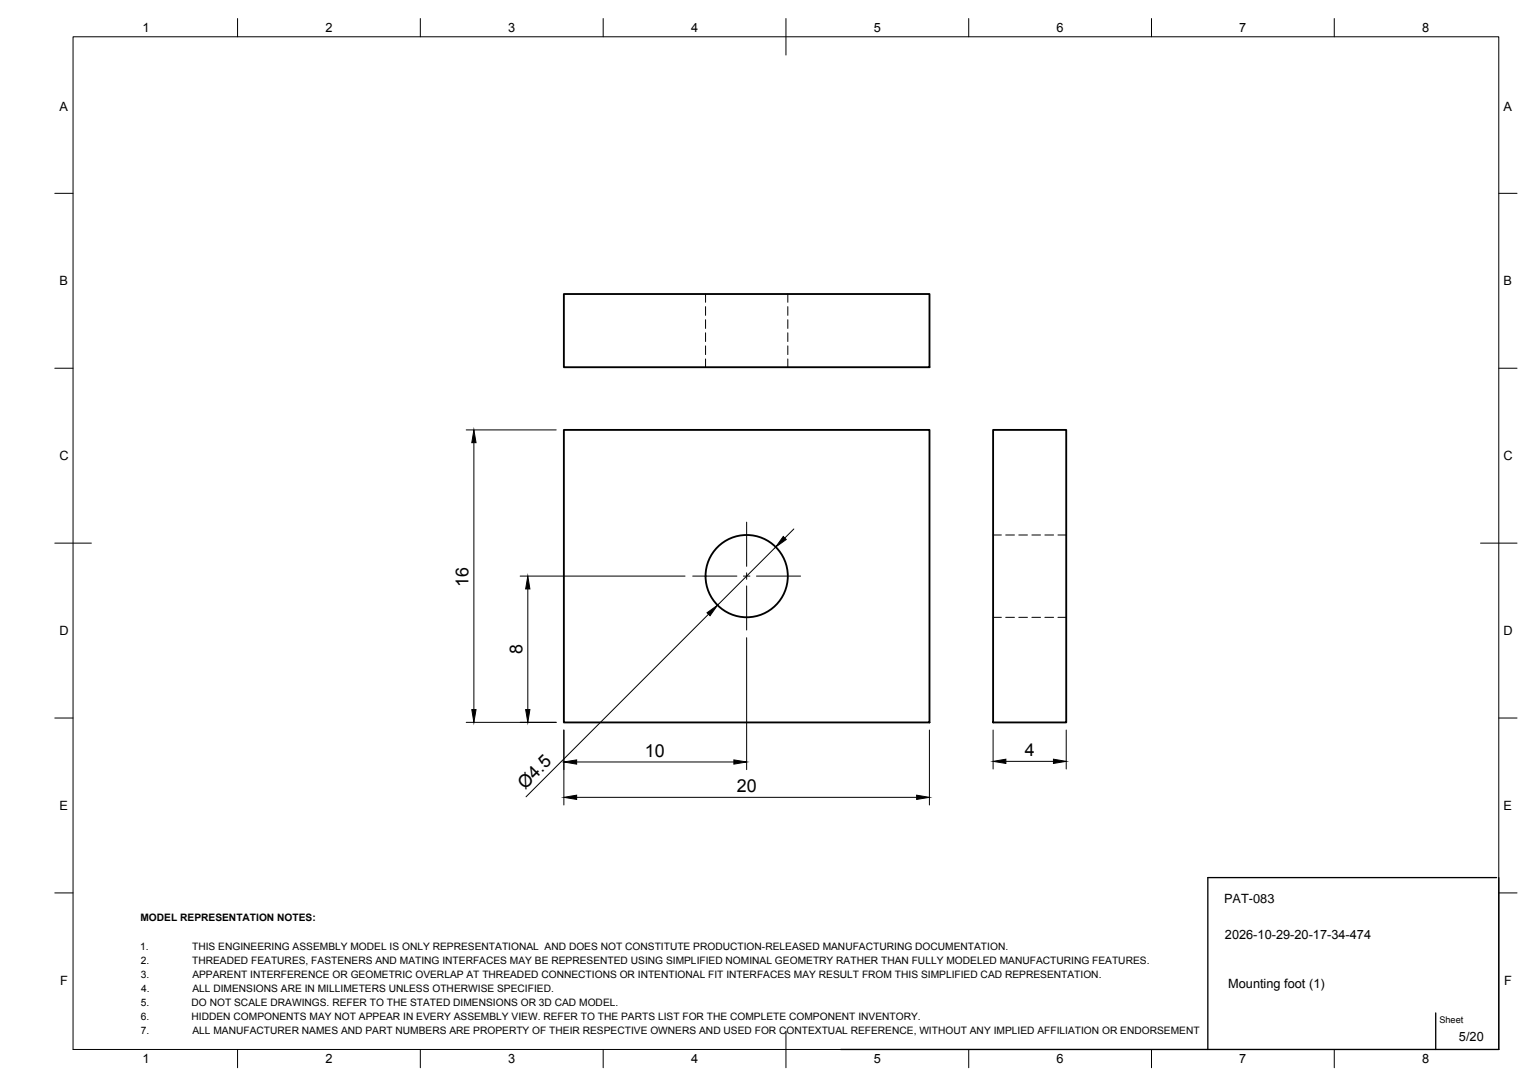
ISO-10303-21;
HEADER;
/* Generated by software containing ST-Developer
 * from STEP Tools, Inc. (www.steptools.com) 
 */

FILE_DESCRIPTION(
/* description */ ('PAT-083'),
/* implementation_level */ '2;1');

FILE_NAME(
/* name */ 'Mounting foot (1).step',
/* time_stamp */ '2026-10-29T20:18:00-07:00',
/* author */ (''),
/* organization */ (''),
/* preprocessor_version */ 'ST-DEVELOPER v20.2',
/* originating_system */ 'Autodesk Translation Framework v15.17.0.0',
/* authorisation */ '');

FILE_SCHEMA (('AUTOMOTIVE_DESIGN { 1 0 10303 214 3 1 1 }'));
ENDSEC;

DATA;
#10=MECHANICAL_DESIGN_GEOMETRIC_PRESENTATION_REPRESENTATION('',(#231),#8428);
#183=SHAPE_REPRESENTATION_RELATIONSHIP('SRR','None',#8517,#207);
#207=ADVANCED_BREP_SHAPE_REPRESENTATION('',(#255),#8406);
#231=STYLED_ITEM('',(#8698),#255);
#255=MANIFOLD_SOLID_BREP('Body1',#3677);
#281=FACE_BOUND('',#755,.T.);
#282=FACE_BOUND('',#757,.T.);
#368=PLANE('',#3994);
#369=PLANE('',#3995);
#370=PLANE('',#3996);
#371=PLANE('',#3997);
#372=PLANE('',#3998);
#373=PLANE('',#3999);
#510=FACE_OUTER_BOUND('',#749,.T.);
#511=FACE_OUTER_BOUND('',#750,.T.);
#512=FACE_OUTER_BOUND('',#751,.T.);
#513=FACE_OUTER_BOUND('',#752,.T.);
#514=FACE_OUTER_BOUND('',#753,.T.);
#515=FACE_OUTER_BOUND('',#754,.T.);
#516=FACE_OUTER_BOUND('',#756,.T.);
#749=EDGE_LOOP('',(#2524,#2525,#2526,#2527));
#750=EDGE_LOOP('',(#2528,#2529,#2530,#2531));
#751=EDGE_LOOP('',(#2532,#2533,#2534,#2535));
#752=EDGE_LOOP('',(#2536,#2537,#2538,#2539));
#753=EDGE_LOOP('',(#2540,#2541,#2542,#2543));
#754=EDGE_LOOP('',(#2544,#2545,#2546,#2547));
#755=EDGE_LOOP('',(#2548));
#756=EDGE_LOOP('',(#2549,#2550,#2551,#2552));
#757=EDGE_LOOP('',(#2553));
#1069=LINE('',#5698,#1313);
#1070=LINE('',#5703,#1314);
#1071=LINE('',#5705,#1315);
#1072=LINE('',#5707,#1316);
#1073=LINE('',#5708,#1317);
#1074=LINE('',#5711,#1318);
#1075=LINE('',#5713,#1319);
#1076=LINE('',#5714,#1320);
#1077=LINE('',#5717,#1321);
#1078=LINE('',#5719,#1322);
#1079=LINE('',#5720,#1323);
#1080=LINE('',#5722,#1324);
#1081=LINE('',#5723,#1325);
#1313=VECTOR('',#4517,0.225);
#1314=VECTOR('',#4522,1.);
#1315=VECTOR('',#4523,1.);
#1316=VECTOR('',#4524,1.);
#1317=VECTOR('',#4525,1.);
#1318=VECTOR('',#4528,1.);
#1319=VECTOR('',#4529,1.);
#1320=VECTOR('',#4530,1.);
#1321=VECTOR('',#4533,1.);
#1322=VECTOR('',#4534,1.);
#1323=VECTOR('',#4535,1.);
#1324=VECTOR('',#4538,1.);
#1325=VECTOR('',#4539,1.);
#1536=CIRCLE('',#3992,0.225);
#1537=CIRCLE('',#3993,0.225);
#1735=VERTEX_POINT('',#5695);
#1736=VERTEX_POINT('',#5697);
#1737=VERTEX_POINT('',#5701);
#1738=VERTEX_POINT('',#5702);
#1739=VERTEX_POINT('',#5704);
#1740=VERTEX_POINT('',#5706);
#1741=VERTEX_POINT('',#5710);
#1742=VERTEX_POINT('',#5712);
#1743=VERTEX_POINT('',#5716);
#1744=VERTEX_POINT('',#5718);
#2038=EDGE_CURVE('',#1735,#1735,#1536,.T.);
#2039=EDGE_CURVE('',#1735,#1736,#1069,.T.);
#2040=EDGE_CURVE('',#1736,#1736,#1537,.T.);
#2041=EDGE_CURVE('',#1737,#1738,#1070,.T.);
#2042=EDGE_CURVE('',#1738,#1739,#1071,.T.);
#2043=EDGE_CURVE('',#1740,#1739,#1072,.T.);
#2044=EDGE_CURVE('',#1737,#1740,#1073,.T.);
#2045=EDGE_CURVE('',#1741,#1737,#1074,.T.);
#2046=EDGE_CURVE('',#1742,#1740,#1075,.T.);
#2047=EDGE_CURVE('',#1741,#1742,#1076,.T.);
#2048=EDGE_CURVE('',#1743,#1741,#1077,.T.);
#2049=EDGE_CURVE('',#1744,#1742,#1078,.T.);
#2050=EDGE_CURVE('',#1743,#1744,#1079,.T.);
#2051=EDGE_CURVE('',#1738,#1743,#1080,.T.);
#2052=EDGE_CURVE('',#1739,#1744,#1081,.T.);
#2524=ORIENTED_EDGE('',*,*,#2038,.F.);
#2525=ORIENTED_EDGE('',*,*,#2039,.T.);
#2526=ORIENTED_EDGE('',*,*,#2040,.F.);
#2527=ORIENTED_EDGE('',*,*,#2039,.F.);
#2528=ORIENTED_EDGE('',*,*,#2041,.T.);
#2529=ORIENTED_EDGE('',*,*,#2042,.T.);
#2530=ORIENTED_EDGE('',*,*,#2043,.F.);
#2531=ORIENTED_EDGE('',*,*,#2044,.F.);
#2532=ORIENTED_EDGE('',*,*,#2045,.T.);
#2533=ORIENTED_EDGE('',*,*,#2044,.T.);
#2534=ORIENTED_EDGE('',*,*,#2046,.F.);
#2535=ORIENTED_EDGE('',*,*,#2047,.F.);
#2536=ORIENTED_EDGE('',*,*,#2048,.T.);
#2537=ORIENTED_EDGE('',*,*,#2047,.T.);
#2538=ORIENTED_EDGE('',*,*,#2049,.F.);
#2539=ORIENTED_EDGE('',*,*,#2050,.F.);
#2540=ORIENTED_EDGE('',*,*,#2051,.T.);
#2541=ORIENTED_EDGE('',*,*,#2050,.T.);
#2542=ORIENTED_EDGE('',*,*,#2052,.F.);
#2543=ORIENTED_EDGE('',*,*,#2042,.F.);
#2544=ORIENTED_EDGE('',*,*,#2052,.T.);
#2545=ORIENTED_EDGE('',*,*,#2049,.T.);
#2546=ORIENTED_EDGE('',*,*,#2046,.T.);
#2547=ORIENTED_EDGE('',*,*,#2043,.T.);
#2548=ORIENTED_EDGE('',*,*,#2040,.T.);
#2549=ORIENTED_EDGE('',*,*,#2051,.F.);
#2550=ORIENTED_EDGE('',*,*,#2041,.F.);
#2551=ORIENTED_EDGE('',*,*,#2045,.F.);
#2552=ORIENTED_EDGE('',*,*,#2048,.F.);
#2553=ORIENTED_EDGE('',*,*,#2038,.T.);
#3367=CYLINDRICAL_SURFACE('',#3991,0.225);
#3457=ADVANCED_FACE('',(#510),#3367,.F.);
#3458=ADVANCED_FACE('',(#511),#368,.T.);
#3459=ADVANCED_FACE('',(#512),#369,.T.);
#3460=ADVANCED_FACE('',(#513),#370,.T.);
#3461=ADVANCED_FACE('',(#514),#371,.T.);
#3462=ADVANCED_FACE('',(#515,#281),#372,.T.);
#3463=ADVANCED_FACE('',(#516,#282),#373,.F.);
#3677=CLOSED_SHELL('',(#3457,#3458,#3459,#3460,#3461,#3462,#3463));
#3990=AXIS2_PLACEMENT_3D('',#5693,#4511,#4512);
#3991=AXIS2_PLACEMENT_3D('',#5694,#4513,#4514);
#3992=AXIS2_PLACEMENT_3D('',#5696,#4515,#4516);
#3993=AXIS2_PLACEMENT_3D('',#5699,#4518,#4519);
#3994=AXIS2_PLACEMENT_3D('',#5700,#4520,#4521);
#3995=AXIS2_PLACEMENT_3D('',#5709,#4526,#4527);
#3996=AXIS2_PLACEMENT_3D('',#5715,#4531,#4532);
#3997=AXIS2_PLACEMENT_3D('',#5721,#4536,#4537);
#3998=AXIS2_PLACEMENT_3D('',#5724,#4540,#4541);
#3999=AXIS2_PLACEMENT_3D('',#5725,#4542,#4543);
#4511=DIRECTION('axis',(0.,0.,1.));
#4512=DIRECTION('refdir',(1.,0.,0.));
#4513=DIRECTION('center_axis',(0.,0.,1.));
#4514=DIRECTION('ref_axis',(1.,0.,0.));
#4515=DIRECTION('center_axis',(0.,0.,1.));
#4516=DIRECTION('ref_axis',(1.,0.,0.));
#4517=DIRECTION('',(0.,0.,1.));
#4518=DIRECTION('center_axis',(0.,0.,-1.));
#4519=DIRECTION('ref_axis',(1.,0.,0.));
#4520=DIRECTION('center_axis',(0.,1.,0.));
#4521=DIRECTION('ref_axis',(-1.,0.,0.));
#4522=DIRECTION('',(-1.,0.,0.));
#4523=DIRECTION('',(0.,0.,1.));
#4524=DIRECTION('',(-1.,0.,0.));
#4525=DIRECTION('',(0.,0.,1.));
#4526=DIRECTION('center_axis',(1.,0.,0.));
#4527=DIRECTION('ref_axis',(0.,1.,0.));
#4528=DIRECTION('',(0.,1.,0.));
#4529=DIRECTION('',(0.,1.,0.));
#4530=DIRECTION('',(0.,0.,1.));
#4531=DIRECTION('center_axis',(0.,-1.,0.));
#4532=DIRECTION('ref_axis',(1.,0.,0.));
#4533=DIRECTION('',(1.,0.,0.));
#4534=DIRECTION('',(1.,0.,0.));
#4535=DIRECTION('',(0.,0.,1.));
#4536=DIRECTION('center_axis',(-1.,0.,0.));
#4537=DIRECTION('ref_axis',(0.,-1.,0.));
#4538=DIRECTION('',(0.,-1.,0.));
#4539=DIRECTION('',(0.,-1.,0.));
#4540=DIRECTION('center_axis',(0.,0.,1.));
#4541=DIRECTION('ref_axis',(1.,0.,0.));
#4542=DIRECTION('center_axis',(0.,0.,1.));
#4543=DIRECTION('ref_axis',(1.,0.,0.));
#5693=CARTESIAN_POINT('',(0.,0.,0.));
#5694=CARTESIAN_POINT('Origin',(0.,3.,0.5));
#5695=CARTESIAN_POINT('',(-0.225,3.,0.6));
#5696=CARTESIAN_POINT('Origin',(0.,3.,0.6));
#5697=CARTESIAN_POINT('',(-0.225,3.,1.));
#5698=CARTESIAN_POINT('',(-0.225,3.,0.5));
#5699=CARTESIAN_POINT('Origin',(0.,3.,1.));
#5700=CARTESIAN_POINT('Origin',(1.,3.8,0.6));
#5701=CARTESIAN_POINT('',(1.,3.8,0.6));
#5702=CARTESIAN_POINT('',(-1.,3.8,0.6));
#5703=CARTESIAN_POINT('',(1.,3.8,0.6));
#5704=CARTESIAN_POINT('',(-1.,3.8,1.));
#5705=CARTESIAN_POINT('',(-1.,3.8,0.6));
#5706=CARTESIAN_POINT('',(1.,3.8,1.));
#5707=CARTESIAN_POINT('',(1.,3.8,1.));
#5708=CARTESIAN_POINT('',(1.,3.8,0.6));
#5709=CARTESIAN_POINT('Origin',(1.,2.2,0.6));
#5710=CARTESIAN_POINT('',(1.,2.2,0.6));
#5711=CARTESIAN_POINT('',(1.,2.2,0.6));
#5712=CARTESIAN_POINT('',(1.,2.2,1.));
#5713=CARTESIAN_POINT('',(1.,2.2,1.));
#5714=CARTESIAN_POINT('',(1.,2.2,0.6));
#5715=CARTESIAN_POINT('Origin',(-1.,2.2,0.6));
#5716=CARTESIAN_POINT('',(-1.,2.2,0.6));
#5717=CARTESIAN_POINT('',(-1.,2.2,0.6));
#5718=CARTESIAN_POINT('',(-1.,2.2,1.));
#5719=CARTESIAN_POINT('',(-1.,2.2,1.));
#5720=CARTESIAN_POINT('',(-1.,2.2,0.6));
#5721=CARTESIAN_POINT('Origin',(-1.,3.8,0.6));
#5722=CARTESIAN_POINT('',(-1.,3.8,0.6));
#5723=CARTESIAN_POINT('',(-1.,3.8,1.));
#5724=CARTESIAN_POINT('Origin',(0.,3.,1.));
#5725=CARTESIAN_POINT('Origin',(0.,3.,0.6));
#8380=UNCERTAINTY_MEASURE_WITH_UNIT(LENGTH_MEASURE(0.001),#8429,
'DISTANCE_ACCURACY_VALUE',
'Maximum model space distance between geometric entities at asserted c
onnectivities');
#8402=UNCERTAINTY_MEASURE_WITH_UNIT(LENGTH_MEASURE(0.001),#8429,
'DISTANCE_ACCURACY_VALUE',
'Maximum model space distance between geometric entities at asserted c
onnectivities');
#8406=(
GEOMETRIC_REPRESENTATION_CONTEXT(3)
GLOBAL_UNCERTAINTY_ASSIGNED_CONTEXT((#8380))
GLOBAL_UNIT_ASSIGNED_CONTEXT((#8429,#8431,#8432))
REPRESENTATION_CONTEXT('','3D')
);
#8428=(
GEOMETRIC_REPRESENTATION_CONTEXT(3)
GLOBAL_UNCERTAINTY_ASSIGNED_CONTEXT((#8402))
GLOBAL_UNIT_ASSIGNED_CONTEXT((#8429,#8431,#8432))
REPRESENTATION_CONTEXT('','3D')
);
#8429=(
LENGTH_UNIT()
NAMED_UNIT(*)
SI_UNIT(.CENTI.,.METRE.)
);
#8431=(
NAMED_UNIT(*)
PLANE_ANGLE_UNIT()
SI_UNIT($,.RADIAN.)
);
#8432=(
NAMED_UNIT(*)
SI_UNIT($,.STERADIAN.)
SOLID_ANGLE_UNIT()
);
#8436=SHAPE_DEFINITION_REPRESENTATION(#8461,#8517);
#8461=PRODUCT_DEFINITION_SHAPE('',$,#8543);
#8517=SHAPE_REPRESENTATION('',(#3990),#8406);
#8539=PRODUCT_DEFINITION_CONTEXT('part definition',#8616,'design');
#8543=PRODUCT_DEFINITION('Mounting foot (1)','Mounting foot (1)',
#8568,#8539);
#8568=PRODUCT_DEFINITION_FORMATION('',$,#8621);
#8616=APPLICATION_CONTEXT(
'Core Data for Automotive Mechanical Design Process');
#8617=PRODUCT_CONTEXT('part definition',#8616,'mechanical');
#8621=PRODUCT('Mounting foot (1)','Mounting foot (1)',
'Mounting foot (1)',(#8617));
#8692=COLOUR_RGB('Sky Blue',0.24,0.69,0.87);
#8693=FILL_AREA_STYLE_COLOUR('',#8692);
#8694=FILL_AREA_STYLE('',(#8693));
#8695=SURFACE_STYLE_FILL_AREA(#8694);
#8696=SURFACE_SIDE_STYLE('',(#8695));
#8697=SURFACE_STYLE_USAGE(.BOTH.,#8696);
#8698=PRESENTATION_STYLE_ASSIGNMENT((#8697));
ENDSEC;
END-ISO-10303-21;
